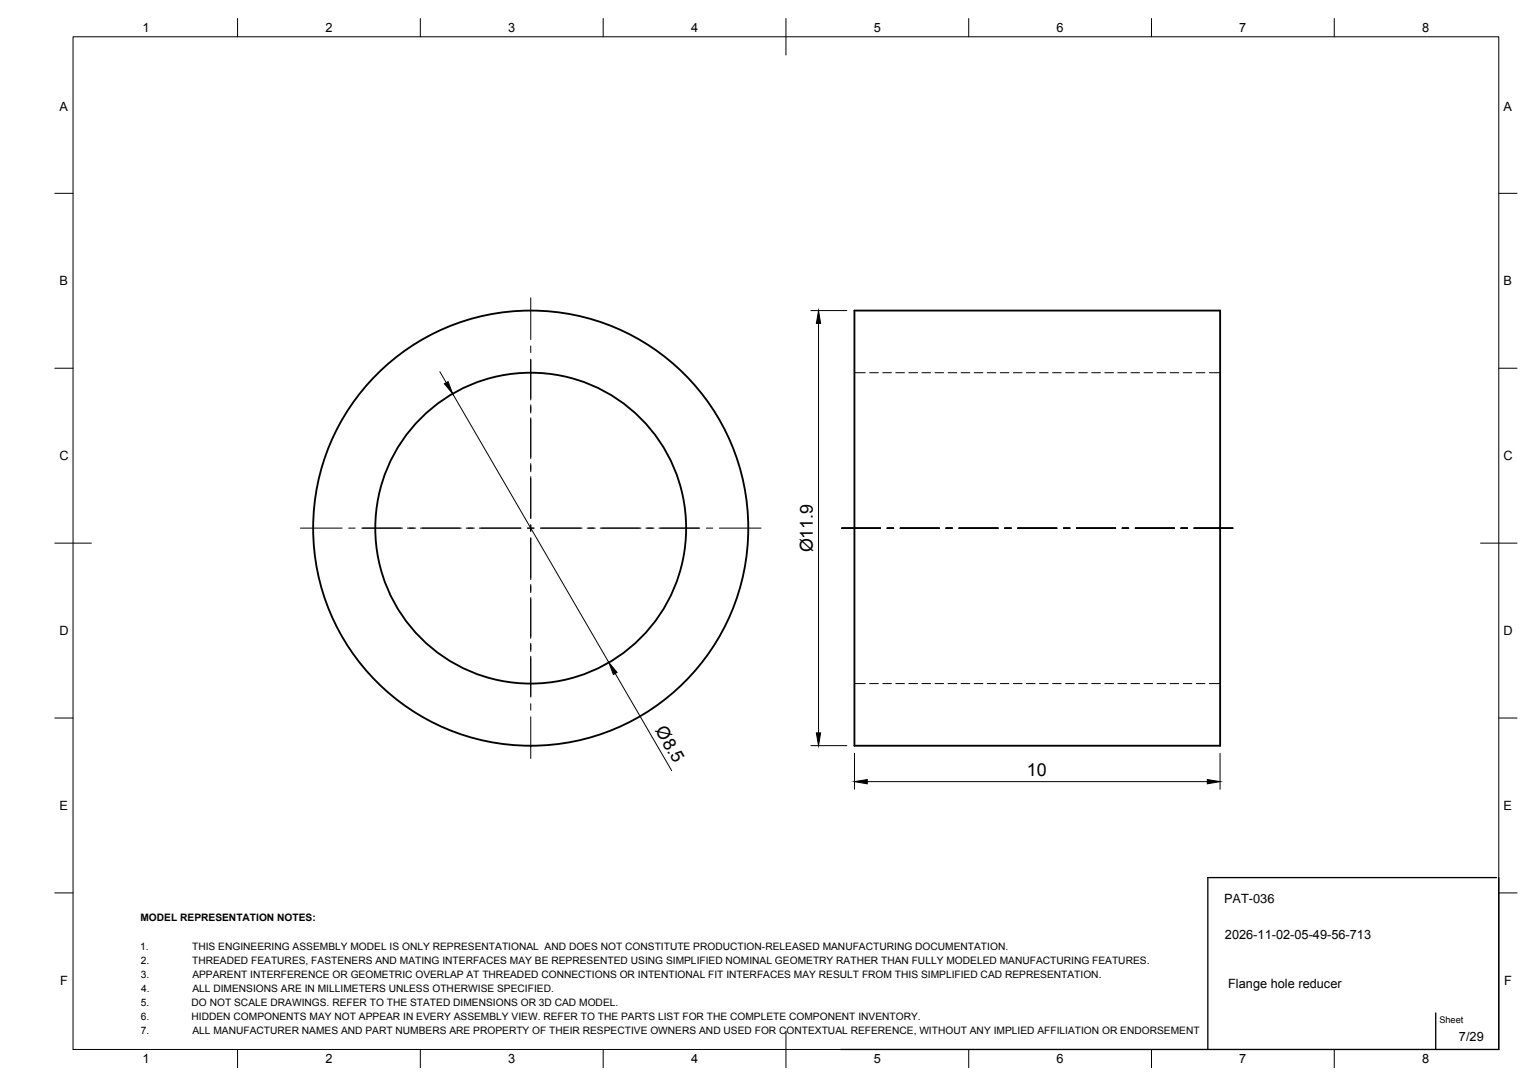
ISO-10303-21;
HEADER;
/* Generated by software containing ST-Developer
 * from STEP Tools, Inc. (www.steptools.com) 
 */

FILE_DESCRIPTION(
/* description */ ('Flange-mounted spindle'),
/* implementation_level */ '2;1');

FILE_NAME(
/* name */ 'Flange hole reducer.step',
/* time_stamp */ '2026-10-27T10:49:51-07:00',
/* author */ (''),
/* organization */ (''),
/* preprocessor_version */ 'ST-DEVELOPER v20.2',
/* originating_system */ 'Autodesk Translation Framework v15.17.0.0',
/* authorisation */ '');

FILE_SCHEMA (('AUTOMOTIVE_DESIGN { 1 0 10303 214 3 1 1 }'));
ENDSEC;

DATA;
#10=MECHANICAL_DESIGN_GEOMETRIC_PRESENTATION_REPRESENTATION('',(#340),#11764);
#286=SHAPE_REPRESENTATION_RELATIONSHIP('SRR','None',#11882,#313);
#313=ADVANCED_BREP_SHAPE_REPRESENTATION('',(#368),#11737);
#340=STYLED_ITEM('',(#12113),#368);
#368=MANIFOLD_SOLID_BREP('Body1',#6132);
#409=FACE_BOUND('',#1063,.T.);
#410=FACE_BOUND('',#1065,.T.);
#520=PLANE('',#6511);
#521=PLANE('',#6512);
#697=FACE_OUTER_BOUND('',#1060,.T.);
#698=FACE_OUTER_BOUND('',#1061,.T.);
#699=FACE_OUTER_BOUND('',#1062,.T.);
#700=FACE_OUTER_BOUND('',#1064,.T.);
#1060=EDGE_LOOP('',(#4119,#4120,#4121,#4122));
#1061=EDGE_LOOP('',(#4123,#4124,#4125,#4126));
#1062=EDGE_LOOP('',(#4127));
#1063=EDGE_LOOP('',(#4128));
#1064=EDGE_LOOP('',(#4129));
#1065=EDGE_LOOP('',(#4130));
#1518=LINE('',#9255,#1940);
#1519=LINE('',#9261,#1941);
#1940=VECTOR('',#7343,0.425);
#1941=VECTOR('',#7350,0.595);
#2341=CIRCLE('',#6506,0.425);
#2342=CIRCLE('',#6507,0.425);
#2343=CIRCLE('',#6509,0.595);
#2344=CIRCLE('',#6510,0.595);
#2687=VERTEX_POINT('',#9252);
#2688=VERTEX_POINT('',#9254);
#2689=VERTEX_POINT('',#9258);
#2690=VERTEX_POINT('',#9260);
#3252=EDGE_CURVE('',#2687,#2687,#2341,.T.);
#3253=EDGE_CURVE('',#2687,#2688,#1518,.T.);
#3254=EDGE_CURVE('',#2688,#2688,#2342,.T.);
#3255=EDGE_CURVE('',#2689,#2689,#2343,.T.);
#3256=EDGE_CURVE('',#2689,#2690,#1519,.T.);
#3257=EDGE_CURVE('',#2690,#2690,#2344,.T.);
#4119=ORIENTED_EDGE('',*,*,#3252,.F.);
#4120=ORIENTED_EDGE('',*,*,#3253,.T.);
#4121=ORIENTED_EDGE('',*,*,#3254,.T.);
#4122=ORIENTED_EDGE('',*,*,#3253,.F.);
#4123=ORIENTED_EDGE('',*,*,#3255,.F.);
#4124=ORIENTED_EDGE('',*,*,#3256,.T.);
#4125=ORIENTED_EDGE('',*,*,#3257,.T.);
#4126=ORIENTED_EDGE('',*,*,#3256,.F.);
#4127=ORIENTED_EDGE('',*,*,#3255,.T.);
#4128=ORIENTED_EDGE('',*,*,#3252,.T.);
#4129=ORIENTED_EDGE('',*,*,#3257,.F.);
#4130=ORIENTED_EDGE('',*,*,#3254,.F.);
#5634=CYLINDRICAL_SURFACE('',#6505,0.425);
#5635=CYLINDRICAL_SURFACE('',#6508,0.595);
#5808=ADVANCED_FACE('',(#697),#5634,.F.);
#5809=ADVANCED_FACE('',(#698),#5635,.T.);
#5810=ADVANCED_FACE('',(#699,#409),#520,.T.);
#5811=ADVANCED_FACE('',(#700,#410),#521,.F.);
#6132=CLOSED_SHELL('',(#5808,#5809,#5810,#5811));
#6504=AXIS2_PLACEMENT_3D('',#9250,#7337,#7338);
#6505=AXIS2_PLACEMENT_3D('',#9251,#7339,#7340);
#6506=AXIS2_PLACEMENT_3D('',#9253,#7341,#7342);
#6507=AXIS2_PLACEMENT_3D('',#9256,#7344,#7345);
#6508=AXIS2_PLACEMENT_3D('',#9257,#7346,#7347);
#6509=AXIS2_PLACEMENT_3D('',#9259,#7348,#7349);
#6510=AXIS2_PLACEMENT_3D('',#9262,#7351,#7352);
#6511=AXIS2_PLACEMENT_3D('',#9263,#7353,#7354);
#6512=AXIS2_PLACEMENT_3D('',#9264,#7355,#7356);
#7337=DIRECTION('axis',(0.,0.,1.));
#7338=DIRECTION('refdir',(1.,0.,0.));
#7339=DIRECTION('center_axis',(0.,1.,0.));
#7340=DIRECTION('ref_axis',(1.,0.,0.));
#7341=DIRECTION('center_axis',(0.,-1.,0.));
#7342=DIRECTION('ref_axis',(1.,0.,0.));
#7343=DIRECTION('',(0.,-1.,0.));
#7344=DIRECTION('center_axis',(0.,-1.,0.));
#7345=DIRECTION('ref_axis',(1.,0.,0.));
#7346=DIRECTION('center_axis',(0.,1.,0.));
#7347=DIRECTION('ref_axis',(1.,0.,0.));
#7348=DIRECTION('center_axis',(0.,1.,0.));
#7349=DIRECTION('ref_axis',(1.,0.,0.));
#7350=DIRECTION('',(0.,-1.,0.));
#7351=DIRECTION('center_axis',(0.,1.,0.));
#7352=DIRECTION('ref_axis',(1.,0.,0.));
#7353=DIRECTION('center_axis',(0.,1.,0.));
#7354=DIRECTION('ref_axis',(1.,0.,0.));
#7355=DIRECTION('center_axis',(0.,1.,0.));
#7356=DIRECTION('ref_axis',(1.,0.,0.));
#9250=CARTESIAN_POINT('',(0.,0.,0.));
#9251=CARTESIAN_POINT('Origin',(-3.2,-0.5,4.8));
#9252=CARTESIAN_POINT('',(-3.625,0.5,4.8));
#9253=CARTESIAN_POINT('Origin',(-3.2,0.5,4.8));
#9254=CARTESIAN_POINT('',(-3.625,-0.5,4.8));
#9255=CARTESIAN_POINT('',(-3.625,-0.5,4.8));
#9256=CARTESIAN_POINT('Origin',(-3.2,-0.5,4.8));
#9257=CARTESIAN_POINT('Origin',(-3.2,-0.5,4.8));
#9258=CARTESIAN_POINT('',(-3.795,0.5,4.8));
#9259=CARTESIAN_POINT('Origin',(-3.2,0.5,4.8));
#9260=CARTESIAN_POINT('',(-3.795,-0.5,4.8));
#9261=CARTESIAN_POINT('',(-3.795,-0.5,4.8));
#9262=CARTESIAN_POINT('Origin',(-3.2,-0.5,4.8));
#9263=CARTESIAN_POINT('Origin',(-3.2,0.5,4.8));
#9264=CARTESIAN_POINT('Origin',(-3.2,-0.5,4.8));
#11705=UNCERTAINTY_MEASURE_WITH_UNIT(LENGTH_MEASURE(0.001),#11765,
'DISTANCE_ACCURACY_VALUE',
'Maximum model space distance between geometric entities at asserted c
onnectivities');
#11732=UNCERTAINTY_MEASURE_WITH_UNIT(LENGTH_MEASURE(0.001),#11765,
'DISTANCE_ACCURACY_VALUE',
'Maximum model space distance between geometric entities at asserted c
onnectivities');
#11737=(
GEOMETRIC_REPRESENTATION_CONTEXT(3)
GLOBAL_UNCERTAINTY_ASSIGNED_CONTEXT((#11705))
GLOBAL_UNIT_ASSIGNED_CONTEXT((#11765,#11767,#11768))
REPRESENTATION_CONTEXT('','3D')
);
#11764=(
GEOMETRIC_REPRESENTATION_CONTEXT(3)
GLOBAL_UNCERTAINTY_ASSIGNED_CONTEXT((#11732))
GLOBAL_UNIT_ASSIGNED_CONTEXT((#11765,#11767,#11768))
REPRESENTATION_CONTEXT('','3D')
);
#11765=(
LENGTH_UNIT()
NAMED_UNIT(*)
SI_UNIT(.CENTI.,.METRE.)
);
#11767=(
NAMED_UNIT(*)
PLANE_ANGLE_UNIT()
SI_UNIT($,.RADIAN.)
);
#11768=(
NAMED_UNIT(*)
SI_UNIT($,.STERADIAN.)
SOLID_ANGLE_UNIT()
);
#11773=SHAPE_DEFINITION_REPRESENTATION(#11804,#11882);
#11804=PRODUCT_DEFINITION_SHAPE('',$,#11914);
#11882=SHAPE_REPRESENTATION('',(#6504),#11737);
#11909=PRODUCT_DEFINITION_CONTEXT('part definition',#12004,'design');
#11914=PRODUCT_DEFINITION('Flange hole reducer','Flange hole reducer',#11945,
#11909);
#11945=PRODUCT_DEFINITION_FORMATION('',$,#12010);
#12004=APPLICATION_CONTEXT(
'Core Data for Automotive Mechanical Design Process');
#12005=PRODUCT_CONTEXT('part definition',#12004,'mechanical');
#12010=PRODUCT('Flange hole reducer','Flange hole reducer',
'Flange hole reducer',(#12005));
#12107=COLOUR_RGB('Off White',0.89,0.88,0.83);
#12108=FILL_AREA_STYLE_COLOUR('',#12107);
#12109=FILL_AREA_STYLE('',(#12108));
#12110=SURFACE_STYLE_FILL_AREA(#12109);
#12111=SURFACE_SIDE_STYLE('',(#12110));
#12112=SURFACE_STYLE_USAGE(.BOTH.,#12111);
#12113=PRESENTATION_STYLE_ASSIGNMENT((#12112));
ENDSEC;
END-ISO-10303-21;
